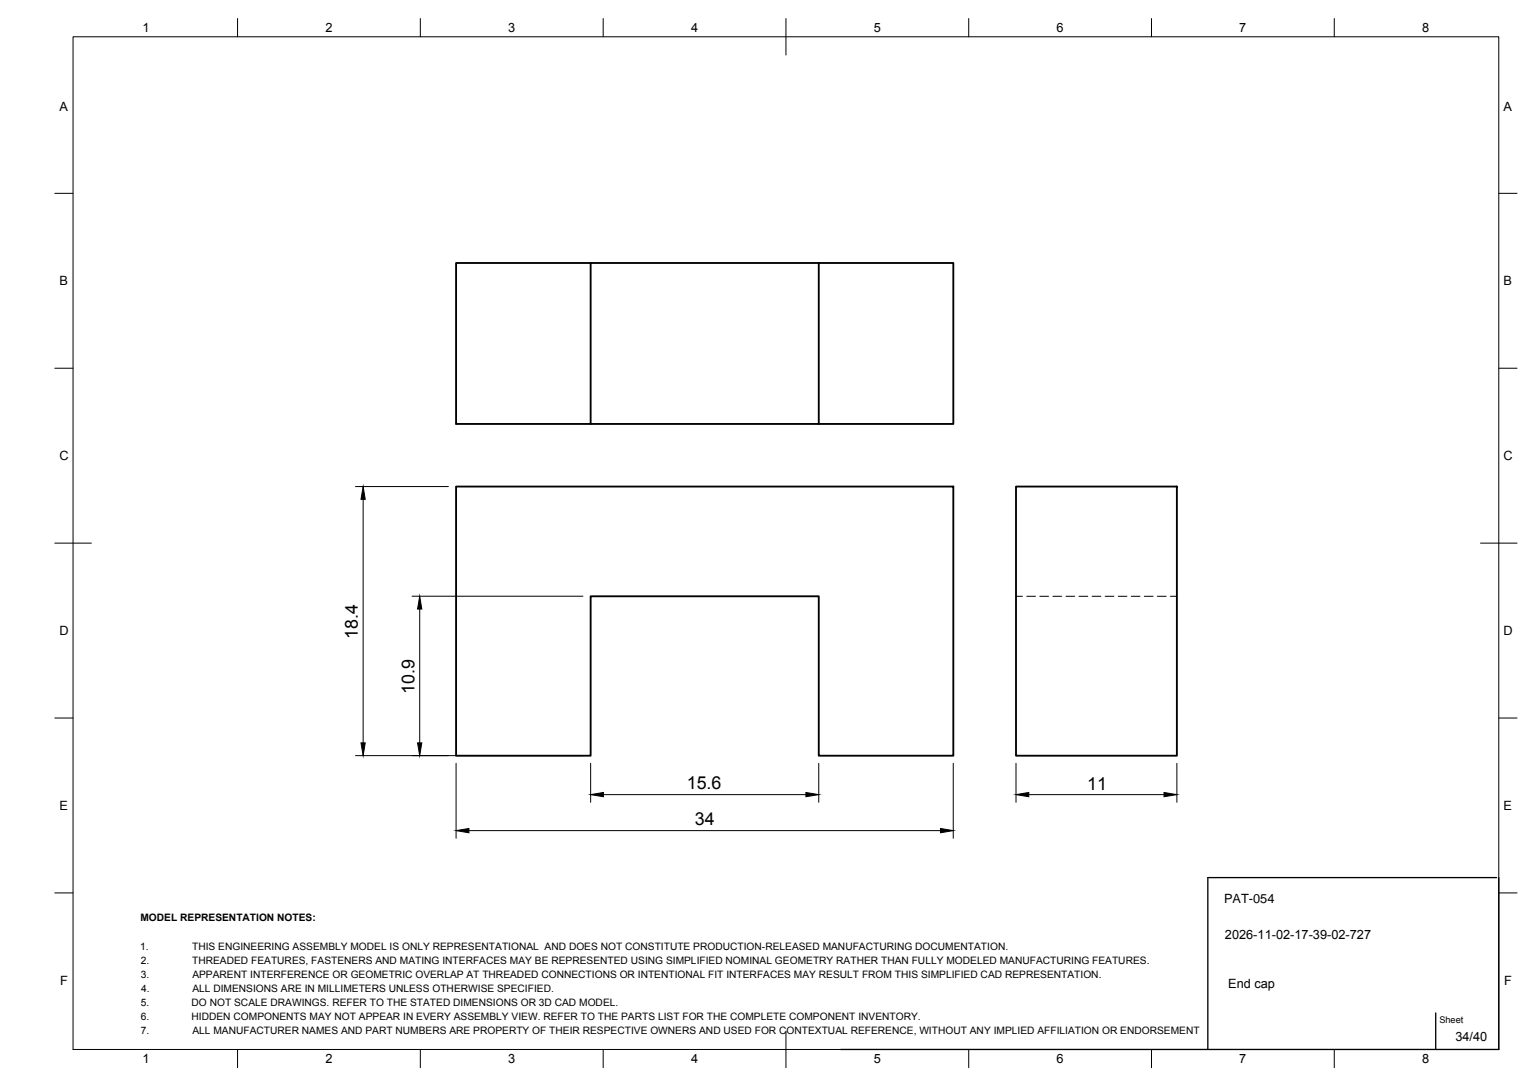
ISO-10303-21;
HEADER;
/* Generated by software containing ST-Developer
 * from STEP Tools, Inc. (www.steptools.com) 
 */

FILE_DESCRIPTION(
/* description */ ('PAT-054'),
/* implementation_level */ '2;1');

FILE_NAME(
/* name */ 'End cap.step',
/* time_stamp */ '2026-10-29T16:38:13-07:00',
/* author */ (''),
/* organization */ (''),
/* preprocessor_version */ 'ST-DEVELOPER v20.2',
/* originating_system */ 'Autodesk Translation Framework v15.17.0.0',
/* authorisation */ '');

FILE_SCHEMA (('AUTOMOTIVE_DESIGN { 1 0 10303 214 3 1 1 }'));
ENDSEC;

DATA;
#10=MECHANICAL_DESIGN_GEOMETRIC_PRESENTATION_REPRESENTATION('',(#942),#33981);
#839=SHAPE_REPRESENTATION_RELATIONSHIP('SRR','None',#34216,#883);
#883=ADVANCED_BREP_SHAPE_REPRESENTATION('',(#1000),#33964);
#942=STYLED_ITEM('',(#34531),#1000);
#1000=MANIFOLD_SOLID_BREP('Body1',#13054);
#1465=PLANE('',#14376);
#1466=PLANE('',#14377);
#1467=PLANE('',#14378);
#1468=PLANE('',#14379);
#1469=PLANE('',#14380);
#1470=PLANE('',#14381);
#1471=PLANE('',#14382);
#1472=PLANE('',#14383);
#1473=PLANE('',#14384);
#1474=PLANE('',#14385);
#1982=FACE_OUTER_BOUND('',#2882,.T.);
#1983=FACE_OUTER_BOUND('',#2883,.T.);
#1984=FACE_OUTER_BOUND('',#2884,.T.);
#1985=FACE_OUTER_BOUND('',#2885,.T.);
#1986=FACE_OUTER_BOUND('',#2886,.T.);
#1987=FACE_OUTER_BOUND('',#2887,.T.);
#1988=FACE_OUTER_BOUND('',#2888,.T.);
#1989=FACE_OUTER_BOUND('',#2889,.T.);
#1990=FACE_OUTER_BOUND('',#2890,.T.);
#1991=FACE_OUTER_BOUND('',#2891,.T.);
#2882=EDGE_LOOP('',(#10421,#10422,#10423,#10424));
#2883=EDGE_LOOP('',(#10425,#10426,#10427,#10428));
#2884=EDGE_LOOP('',(#10429,#10430,#10431,#10432));
#2885=EDGE_LOOP('',(#10433,#10434,#10435,#10436));
#2886=EDGE_LOOP('',(#10437,#10438,#10439,#10440));
#2887=EDGE_LOOP('',(#10441,#10442,#10443,#10444));
#2888=EDGE_LOOP('',(#10445,#10446,#10447,#10448));
#2889=EDGE_LOOP('',(#10449,#10450,#10451,#10452));
#2890=EDGE_LOOP('',(#10453,#10454,#10455,#10456,#10457,#10458,#10459,#10460));
#2891=EDGE_LOOP('',(#10461,#10462,#10463,#10464,#10465,#10466,#10467,#10468));
#3806=LINE('',#21199,#4740);
#3807=LINE('',#21201,#4741);
#3808=LINE('',#21203,#4742);
#3809=LINE('',#21204,#4743);
#3810=LINE('',#21207,#4744);
#3811=LINE('',#21209,#4745);
#3812=LINE('',#21210,#4746);
#3813=LINE('',#21213,#4747);
#3814=LINE('',#21215,#4748);
#3815=LINE('',#21216,#4749);
#3816=LINE('',#21219,#4750);
#3817=LINE('',#21221,#4751);
#3818=LINE('',#21222,#4752);
#3819=LINE('',#21225,#4753);
#3820=LINE('',#21227,#4754);
#3821=LINE('',#21228,#4755);
#3822=LINE('',#21231,#4756);
#3823=LINE('',#21233,#4757);
#3824=LINE('',#21234,#4758);
#3825=LINE('',#21237,#4759);
#3826=LINE('',#21239,#4760);
#3827=LINE('',#21240,#4761);
#3828=LINE('',#21242,#4762);
#3829=LINE('',#21243,#4763);
#4740=VECTOR('',#17095,1.);
#4741=VECTOR('',#17096,1.);
#4742=VECTOR('',#17097,1.);
#4743=VECTOR('',#17098,1.);
#4744=VECTOR('',#17101,1.);
#4745=VECTOR('',#17102,1.);
#4746=VECTOR('',#17103,1.);
#4747=VECTOR('',#17106,1.);
#4748=VECTOR('',#17107,1.);
#4749=VECTOR('',#17108,1.);
#4750=VECTOR('',#17111,1.);
#4751=VECTOR('',#17112,1.);
#4752=VECTOR('',#17113,1.);
#4753=VECTOR('',#17116,1.);
#4754=VECTOR('',#17117,1.);
#4755=VECTOR('',#17118,1.);
#4756=VECTOR('',#17121,1.);
#4757=VECTOR('',#17122,1.);
#4758=VECTOR('',#17123,1.);
#4759=VECTOR('',#17126,1.);
#4760=VECTOR('',#17127,1.);
#4761=VECTOR('',#17128,1.);
#4762=VECTOR('',#17131,1.);
#4763=VECTOR('',#17132,1.);
#6230=VERTEX_POINT('',#21197);
#6231=VERTEX_POINT('',#21198);
#6232=VERTEX_POINT('',#21200);
#6233=VERTEX_POINT('',#21202);
#6234=VERTEX_POINT('',#21206);
#6235=VERTEX_POINT('',#21208);
#6236=VERTEX_POINT('',#21212);
#6237=VERTEX_POINT('',#21214);
#6238=VERTEX_POINT('',#21218);
#6239=VERTEX_POINT('',#21220);
#6240=VERTEX_POINT('',#21224);
#6241=VERTEX_POINT('',#21226);
#6242=VERTEX_POINT('',#21230);
#6243=VERTEX_POINT('',#21232);
#6244=VERTEX_POINT('',#21236);
#6245=VERTEX_POINT('',#21238);
#7710=EDGE_CURVE('',#6230,#6231,#3806,.T.);
#7711=EDGE_CURVE('',#6230,#6232,#3807,.T.);
#7712=EDGE_CURVE('',#6233,#6232,#3808,.T.);
#7713=EDGE_CURVE('',#6231,#6233,#3809,.T.);
#7714=EDGE_CURVE('',#6231,#6234,#3810,.T.);
#7715=EDGE_CURVE('',#6235,#6233,#3811,.T.);
#7716=EDGE_CURVE('',#6234,#6235,#3812,.T.);
#7717=EDGE_CURVE('',#6234,#6236,#3813,.T.);
#7718=EDGE_CURVE('',#6237,#6235,#3814,.T.);
#7719=EDGE_CURVE('',#6236,#6237,#3815,.T.);
#7720=EDGE_CURVE('',#6236,#6238,#3816,.T.);
#7721=EDGE_CURVE('',#6239,#6237,#3817,.T.);
#7722=EDGE_CURVE('',#6238,#6239,#3818,.T.);
#7723=EDGE_CURVE('',#6238,#6240,#3819,.T.);
#7724=EDGE_CURVE('',#6241,#6239,#3820,.T.);
#7725=EDGE_CURVE('',#6240,#6241,#3821,.T.);
#7726=EDGE_CURVE('',#6240,#6242,#3822,.T.);
#7727=EDGE_CURVE('',#6243,#6241,#3823,.T.);
#7728=EDGE_CURVE('',#6242,#6243,#3824,.T.);
#7729=EDGE_CURVE('',#6242,#6244,#3825,.T.);
#7730=EDGE_CURVE('',#6245,#6243,#3826,.T.);
#7731=EDGE_CURVE('',#6244,#6245,#3827,.T.);
#7732=EDGE_CURVE('',#6244,#6230,#3828,.T.);
#7733=EDGE_CURVE('',#6232,#6245,#3829,.T.);
#10421=ORIENTED_EDGE('',*,*,#7710,.F.);
#10422=ORIENTED_EDGE('',*,*,#7711,.T.);
#10423=ORIENTED_EDGE('',*,*,#7712,.F.);
#10424=ORIENTED_EDGE('',*,*,#7713,.F.);
#10425=ORIENTED_EDGE('',*,*,#7714,.F.);
#10426=ORIENTED_EDGE('',*,*,#7713,.T.);
#10427=ORIENTED_EDGE('',*,*,#7715,.F.);
#10428=ORIENTED_EDGE('',*,*,#7716,.F.);
#10429=ORIENTED_EDGE('',*,*,#7717,.F.);
#10430=ORIENTED_EDGE('',*,*,#7716,.T.);
#10431=ORIENTED_EDGE('',*,*,#7718,.F.);
#10432=ORIENTED_EDGE('',*,*,#7719,.F.);
#10433=ORIENTED_EDGE('',*,*,#7720,.F.);
#10434=ORIENTED_EDGE('',*,*,#7719,.T.);
#10435=ORIENTED_EDGE('',*,*,#7721,.F.);
#10436=ORIENTED_EDGE('',*,*,#7722,.F.);
#10437=ORIENTED_EDGE('',*,*,#7723,.F.);
#10438=ORIENTED_EDGE('',*,*,#7722,.T.);
#10439=ORIENTED_EDGE('',*,*,#7724,.F.);
#10440=ORIENTED_EDGE('',*,*,#7725,.F.);
#10441=ORIENTED_EDGE('',*,*,#7726,.F.);
#10442=ORIENTED_EDGE('',*,*,#7725,.T.);
#10443=ORIENTED_EDGE('',*,*,#7727,.F.);
#10444=ORIENTED_EDGE('',*,*,#7728,.F.);
#10445=ORIENTED_EDGE('',*,*,#7729,.F.);
#10446=ORIENTED_EDGE('',*,*,#7728,.T.);
#10447=ORIENTED_EDGE('',*,*,#7730,.F.);
#10448=ORIENTED_EDGE('',*,*,#7731,.F.);
#10449=ORIENTED_EDGE('',*,*,#7732,.F.);
#10450=ORIENTED_EDGE('',*,*,#7731,.T.);
#10451=ORIENTED_EDGE('',*,*,#7733,.F.);
#10452=ORIENTED_EDGE('',*,*,#7711,.F.);
#10453=ORIENTED_EDGE('',*,*,#7732,.T.);
#10454=ORIENTED_EDGE('',*,*,#7710,.T.);
#10455=ORIENTED_EDGE('',*,*,#7714,.T.);
#10456=ORIENTED_EDGE('',*,*,#7717,.T.);
#10457=ORIENTED_EDGE('',*,*,#7720,.T.);
#10458=ORIENTED_EDGE('',*,*,#7723,.T.);
#10459=ORIENTED_EDGE('',*,*,#7726,.T.);
#10460=ORIENTED_EDGE('',*,*,#7729,.T.);
#10461=ORIENTED_EDGE('',*,*,#7733,.T.);
#10462=ORIENTED_EDGE('',*,*,#7730,.T.);
#10463=ORIENTED_EDGE('',*,*,#7727,.T.);
#10464=ORIENTED_EDGE('',*,*,#7724,.T.);
#10465=ORIENTED_EDGE('',*,*,#7721,.T.);
#10466=ORIENTED_EDGE('',*,*,#7718,.T.);
#10467=ORIENTED_EDGE('',*,*,#7715,.T.);
#10468=ORIENTED_EDGE('',*,*,#7712,.T.);
#12694=ADVANCED_FACE('',(#1982),#1465,.T.);
#12695=ADVANCED_FACE('',(#1983),#1466,.T.);
#12696=ADVANCED_FACE('',(#1984),#1467,.T.);
#12697=ADVANCED_FACE('',(#1985),#1468,.T.);
#12698=ADVANCED_FACE('',(#1986),#1469,.T.);
#12699=ADVANCED_FACE('',(#1987),#1470,.T.);
#12700=ADVANCED_FACE('',(#1988),#1471,.T.);
#12701=ADVANCED_FACE('',(#1989),#1472,.T.);
#12702=ADVANCED_FACE('',(#1990),#1473,.T.);
#12703=ADVANCED_FACE('',(#1991),#1474,.T.);
#13054=CLOSED_SHELL('',(#12694,#12695,#12696,#12697,#12698,#12699,#12700,
#12701,#12702,#12703));
#14375=AXIS2_PLACEMENT_3D('',#21195,#17091,#17092);
#14376=AXIS2_PLACEMENT_3D('',#21196,#17093,#17094);
#14377=AXIS2_PLACEMENT_3D('',#21205,#17099,#17100);
#14378=AXIS2_PLACEMENT_3D('',#21211,#17104,#17105);
#14379=AXIS2_PLACEMENT_3D('',#21217,#17109,#17110);
#14380=AXIS2_PLACEMENT_3D('',#21223,#17114,#17115);
#14381=AXIS2_PLACEMENT_3D('',#21229,#17119,#17120);
#14382=AXIS2_PLACEMENT_3D('',#21235,#17124,#17125);
#14383=AXIS2_PLACEMENT_3D('',#21241,#17129,#17130);
#14384=AXIS2_PLACEMENT_3D('',#21244,#17133,#17134);
#14385=AXIS2_PLACEMENT_3D('',#21245,#17135,#17136);
#17091=DIRECTION('axis',(0.,0.,1.));
#17092=DIRECTION('refdir',(1.,0.,0.));
#17093=DIRECTION('center_axis',(0.,0.,-1.));
#17094=DIRECTION('ref_axis',(0.,-1.,0.));
#17095=DIRECTION('',(0.,1.,0.));
#17096=DIRECTION('',(-1.,0.,0.));
#17097=DIRECTION('',(0.,-1.,0.));
#17098=DIRECTION('',(-1.,0.,0.));
#17099=DIRECTION('center_axis',(0.,1.,0.));
#17100=DIRECTION('ref_axis',(0.,0.,-1.));
#17101=DIRECTION('',(0.,0.,1.));
#17102=DIRECTION('',(0.,0.,-1.));
#17103=DIRECTION('',(-1.,0.,0.));
#17104=DIRECTION('center_axis',(0.,0.,-1.));
#17105=DIRECTION('ref_axis',(0.,-1.,0.));
#17106=DIRECTION('',(0.,1.,0.));
#17107=DIRECTION('',(0.,-1.,0.));
#17108=DIRECTION('',(-1.,0.,0.));
#17109=DIRECTION('center_axis',(0.,-1.,0.));
#17110=DIRECTION('ref_axis',(0.,0.,1.));
#17111=DIRECTION('',(0.,0.,-1.));
#17112=DIRECTION('',(0.,0.,1.));
#17113=DIRECTION('',(-1.,0.,0.));
#17114=DIRECTION('center_axis',(0.,0.,-1.));
#17115=DIRECTION('ref_axis',(0.,-1.,0.));
#17116=DIRECTION('',(0.,1.,0.));
#17117=DIRECTION('',(0.,-1.,0.));
#17118=DIRECTION('',(-1.,0.,0.));
#17119=DIRECTION('center_axis',(0.,1.,0.));
#17120=DIRECTION('ref_axis',(0.,0.,-1.));
#17121=DIRECTION('',(0.,0.,1.));
#17122=DIRECTION('',(0.,0.,-1.));
#17123=DIRECTION('',(-1.,0.,0.));
#17124=DIRECTION('center_axis',(0.,0.,1.));
#17125=DIRECTION('ref_axis',(0.,1.,0.));
#17126=DIRECTION('',(0.,-1.,0.));
#17127=DIRECTION('',(0.,1.,0.));
#17128=DIRECTION('',(-1.,0.,0.));
#17129=DIRECTION('center_axis',(0.,-1.,0.));
#17130=DIRECTION('ref_axis',(0.,0.,1.));
#17131=DIRECTION('',(0.,0.,-1.));
#17132=DIRECTION('',(0.,0.,1.));
#17133=DIRECTION('center_axis',(1.,0.,0.));
#17134=DIRECTION('ref_axis',(0.,0.,-1.));
#17135=DIRECTION('center_axis',(-1.,0.,0.));
#17136=DIRECTION('ref_axis',(0.,0.,1.));
#21195=CARTESIAN_POINT('',(0.,0.,0.));
#21196=CARTESIAN_POINT('Origin',(-1.97,-0.78,0.46));
#21197=CARTESIAN_POINT('',(-1.97,-1.7,0.46));
#21198=CARTESIAN_POINT('',(-1.97,-0.78,0.46));
#21199=CARTESIAN_POINT('',(-1.97,-1.7,0.46));
#21200=CARTESIAN_POINT('',(-3.07,-1.7,0.46));
#21201=CARTESIAN_POINT('',(-1.97,-1.7,0.46));
#21202=CARTESIAN_POINT('',(-3.07,-0.78,0.46));
#21203=CARTESIAN_POINT('',(-3.07,-1.7,0.46));
#21204=CARTESIAN_POINT('',(-1.97,-0.78,0.46));
#21205=CARTESIAN_POINT('Origin',(-1.97,-0.78,1.55));
#21206=CARTESIAN_POINT('',(-1.97,-0.78,1.55));
#21207=CARTESIAN_POINT('',(-1.97,-0.78,0.46));
#21208=CARTESIAN_POINT('',(-3.07,-0.78,1.55));
#21209=CARTESIAN_POINT('',(-3.07,-0.78,0.46));
#21210=CARTESIAN_POINT('',(-1.97,-0.78,1.55));
#21211=CARTESIAN_POINT('Origin',(-1.97,0.78,1.55));
#21212=CARTESIAN_POINT('',(-1.97,0.78,1.55));
#21213=CARTESIAN_POINT('',(-1.97,-0.78,1.55));
#21214=CARTESIAN_POINT('',(-3.07,0.78,1.55));
#21215=CARTESIAN_POINT('',(-3.07,-0.78,1.55));
#21216=CARTESIAN_POINT('',(-1.97,0.78,1.55));
#21217=CARTESIAN_POINT('Origin',(-1.97,0.78,0.46));
#21218=CARTESIAN_POINT('',(-1.97,0.78,0.46));
#21219=CARTESIAN_POINT('',(-1.97,0.78,1.55));
#21220=CARTESIAN_POINT('',(-3.07,0.78,0.46));
#21221=CARTESIAN_POINT('',(-3.07,0.78,1.55));
#21222=CARTESIAN_POINT('',(-1.97,0.78,0.46));
#21223=CARTESIAN_POINT('Origin',(-1.97,1.7,0.46));
#21224=CARTESIAN_POINT('',(-1.97,1.7,0.46));
#21225=CARTESIAN_POINT('',(-1.97,0.78,0.46));
#21226=CARTESIAN_POINT('',(-3.07,1.7,0.46));
#21227=CARTESIAN_POINT('',(-3.07,0.78,0.46));
#21228=CARTESIAN_POINT('',(-1.97,1.7,0.46));
#21229=CARTESIAN_POINT('Origin',(-1.97,1.7,2.3));
#21230=CARTESIAN_POINT('',(-1.97,1.7,2.3));
#21231=CARTESIAN_POINT('',(-1.97,1.7,0.46));
#21232=CARTESIAN_POINT('',(-3.07,1.7,2.3));
#21233=CARTESIAN_POINT('',(-3.07,1.7,0.46));
#21234=CARTESIAN_POINT('',(-1.97,1.7,2.3));
#21235=CARTESIAN_POINT('Origin',(-1.97,-1.7,2.3));
#21236=CARTESIAN_POINT('',(-1.97,-1.7,2.3));
#21237=CARTESIAN_POINT('',(-1.97,1.7,2.3));
#21238=CARTESIAN_POINT('',(-3.07,-1.7,2.3));
#21239=CARTESIAN_POINT('',(-3.07,1.7,2.3));
#21240=CARTESIAN_POINT('',(-1.97,-1.7,2.3));
#21241=CARTESIAN_POINT('Origin',(-1.97,-1.7,0.46));
#21242=CARTESIAN_POINT('',(-1.97,-1.7,2.3));
#21243=CARTESIAN_POINT('',(-3.07,-1.7,2.3));
#21244=CARTESIAN_POINT('Origin',(-1.97,0.,1.38));
#21245=CARTESIAN_POINT('Origin',(-3.07,0.,1.38));
#33912=UNCERTAINTY_MEASURE_WITH_UNIT(LENGTH_MEASURE(0.001),#33982,
'DISTANCE_ACCURACY_VALUE',
'Maximum model space distance between geometric entities at asserted c
onnectivities');
#33929=UNCERTAINTY_MEASURE_WITH_UNIT(LENGTH_MEASURE(0.001),#33982,
'DISTANCE_ACCURACY_VALUE',
'Maximum model space distance between geometric entities at asserted c
onnectivities');
#33964=(
GEOMETRIC_REPRESENTATION_CONTEXT(3)
GLOBAL_UNCERTAINTY_ASSIGNED_CONTEXT((#33912))
GLOBAL_UNIT_ASSIGNED_CONTEXT((#33982,#33984,#33985))
REPRESENTATION_CONTEXT('','3D')
);
#33981=(
GEOMETRIC_REPRESENTATION_CONTEXT(3)
GLOBAL_UNCERTAINTY_ASSIGNED_CONTEXT((#33929))
GLOBAL_UNIT_ASSIGNED_CONTEXT((#33982,#33984,#33985))
REPRESENTATION_CONTEXT('','3D')
);
#33982=(
LENGTH_UNIT()
NAMED_UNIT(*)
SI_UNIT(.CENTI.,.METRE.)
);
#33984=(
NAMED_UNIT(*)
PLANE_ANGLE_UNIT()
SI_UNIT($,.RADIAN.)
);
#33985=(
NAMED_UNIT(*)
SI_UNIT($,.STERADIAN.)
SOLID_ANGLE_UNIT()
);
#34020=SHAPE_DEFINITION_REPRESENTATION(#34081,#34216);
#34081=PRODUCT_DEFINITION_SHAPE('',$,#34268);
#34216=SHAPE_REPRESENTATION('',(#14375),#33964);
#34233=PRODUCT_DEFINITION_CONTEXT('part definition',#34388,'design');
#34268=PRODUCT_DEFINITION('End cap','End cap',#34319,#34233);
#34319=PRODUCT_DEFINITION_FORMATION('',$,#34424);
#34388=APPLICATION_CONTEXT(
'Core Data for Automotive Mechanical Design Process');
#34389=PRODUCT_CONTEXT('part definition',#34388,'mechanical');
#34424=PRODUCT('End cap','End cap','End cap',(#34389));
#34525=COLOUR_RGB('Off White',0.89,0.88,0.83);
#34526=FILL_AREA_STYLE_COLOUR('',#34525);
#34527=FILL_AREA_STYLE('',(#34526));
#34528=SURFACE_STYLE_FILL_AREA(#34527);
#34529=SURFACE_SIDE_STYLE('',(#34528));
#34530=SURFACE_STYLE_USAGE(.BOTH.,#34529);
#34531=PRESENTATION_STYLE_ASSIGNMENT((#34530));
ENDSEC;
END-ISO-10303-21;
